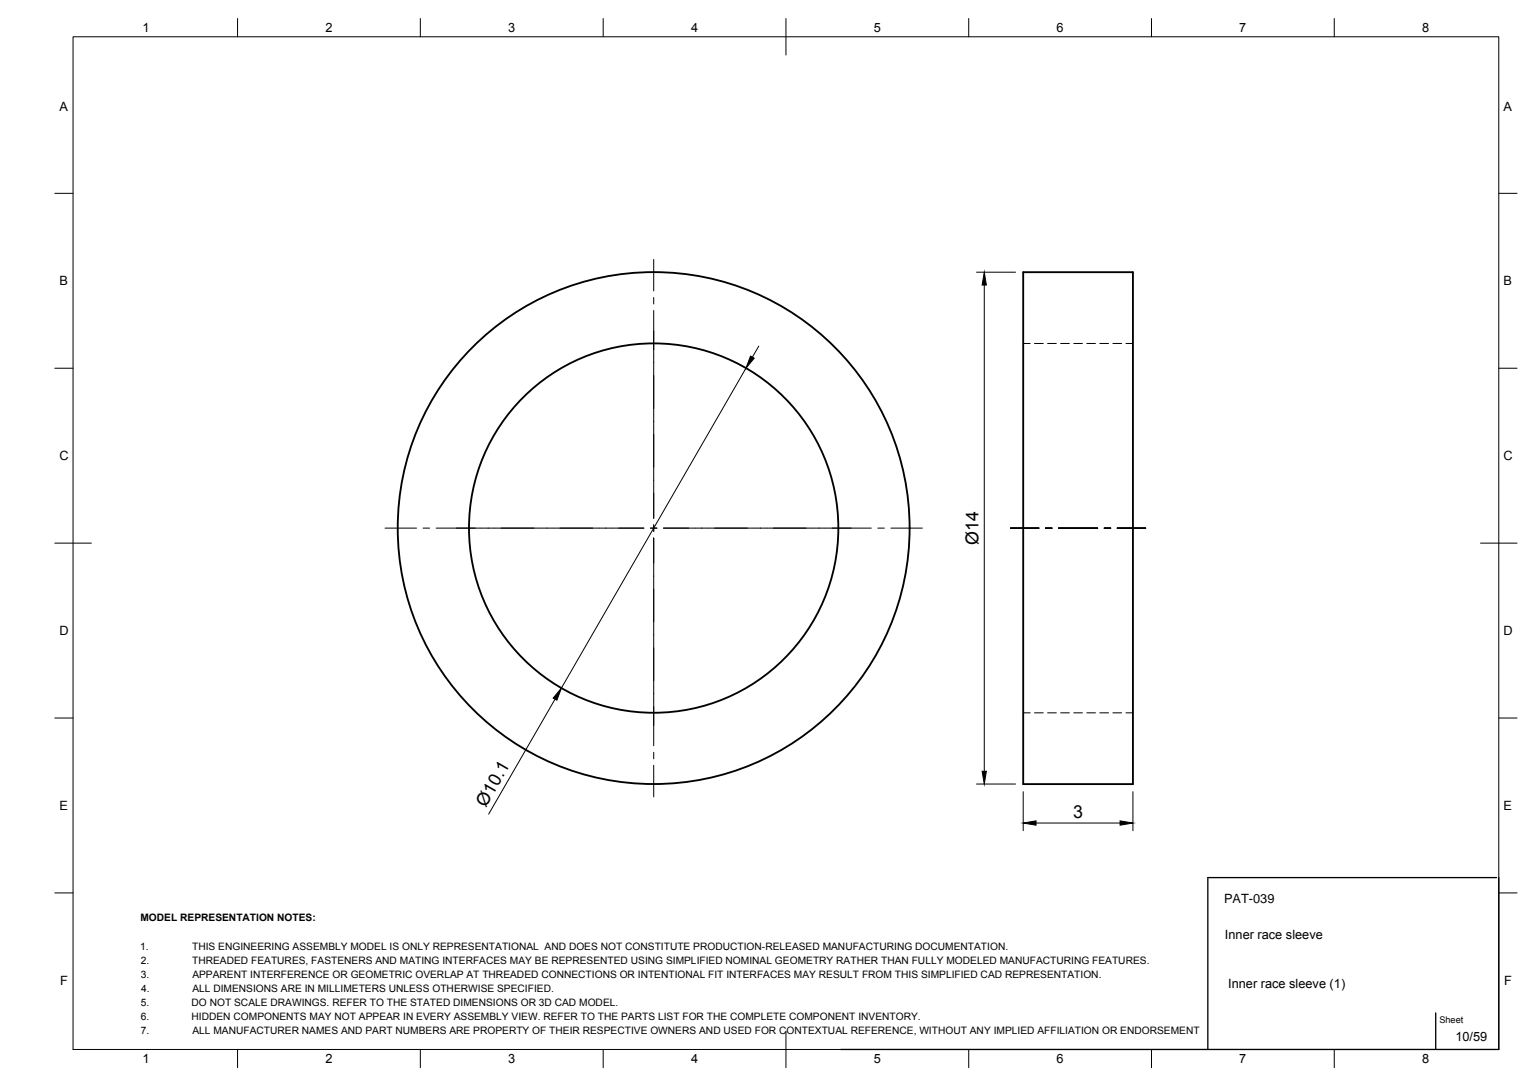
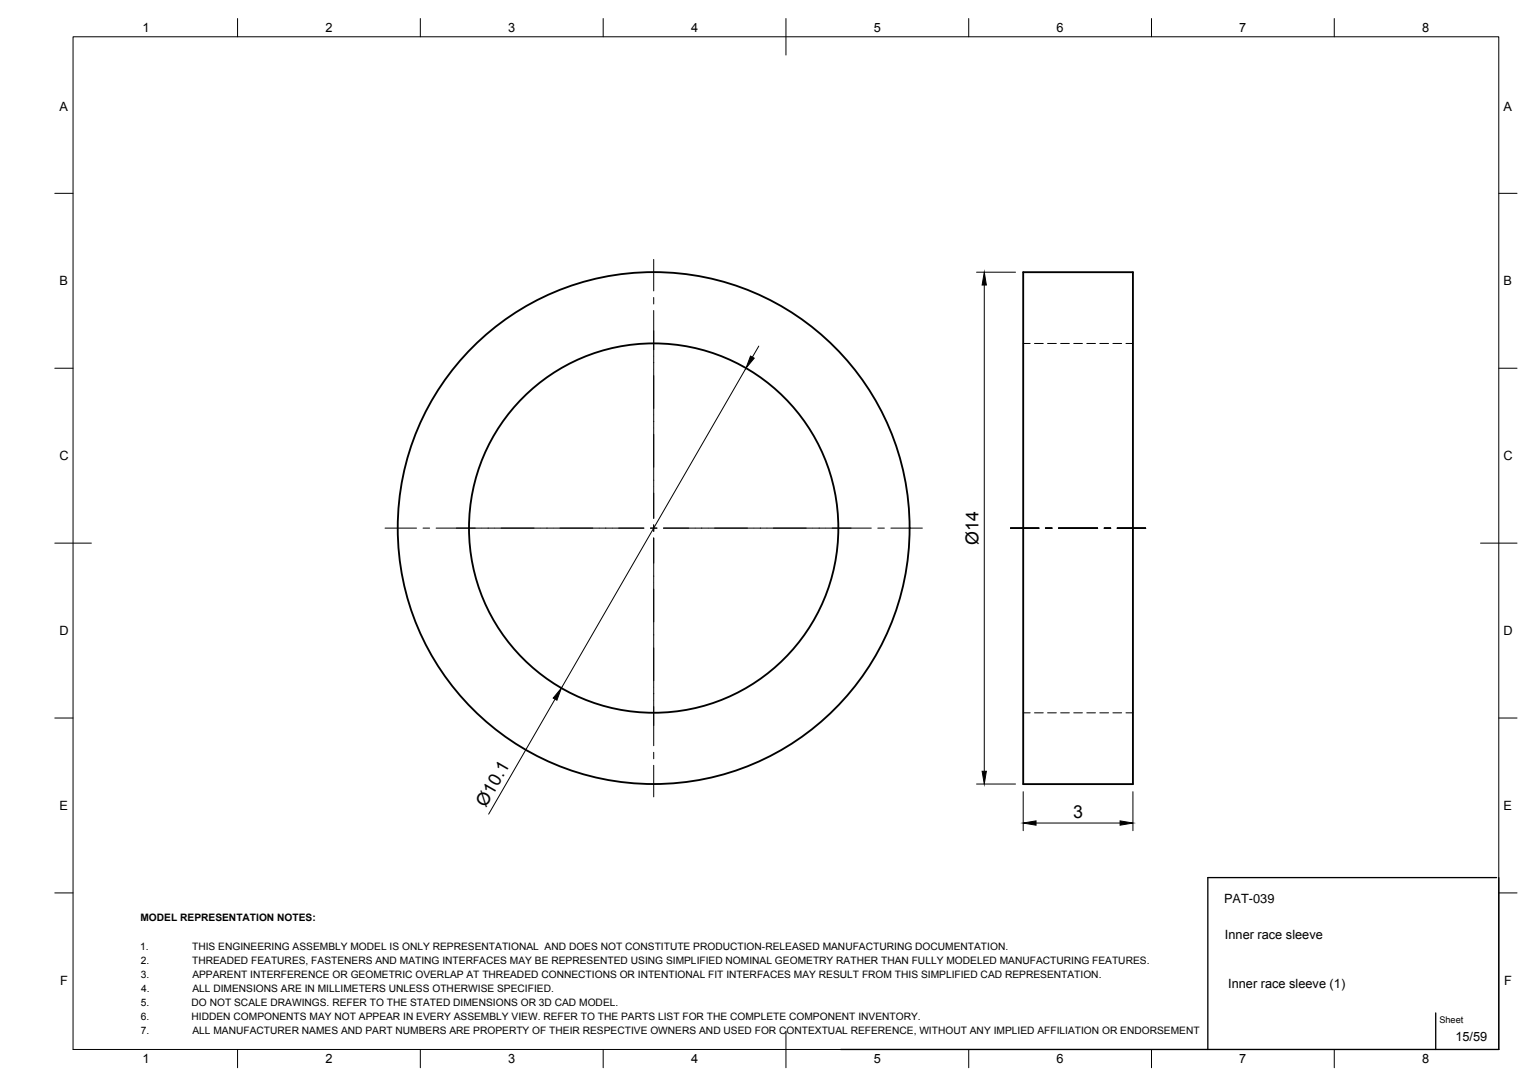
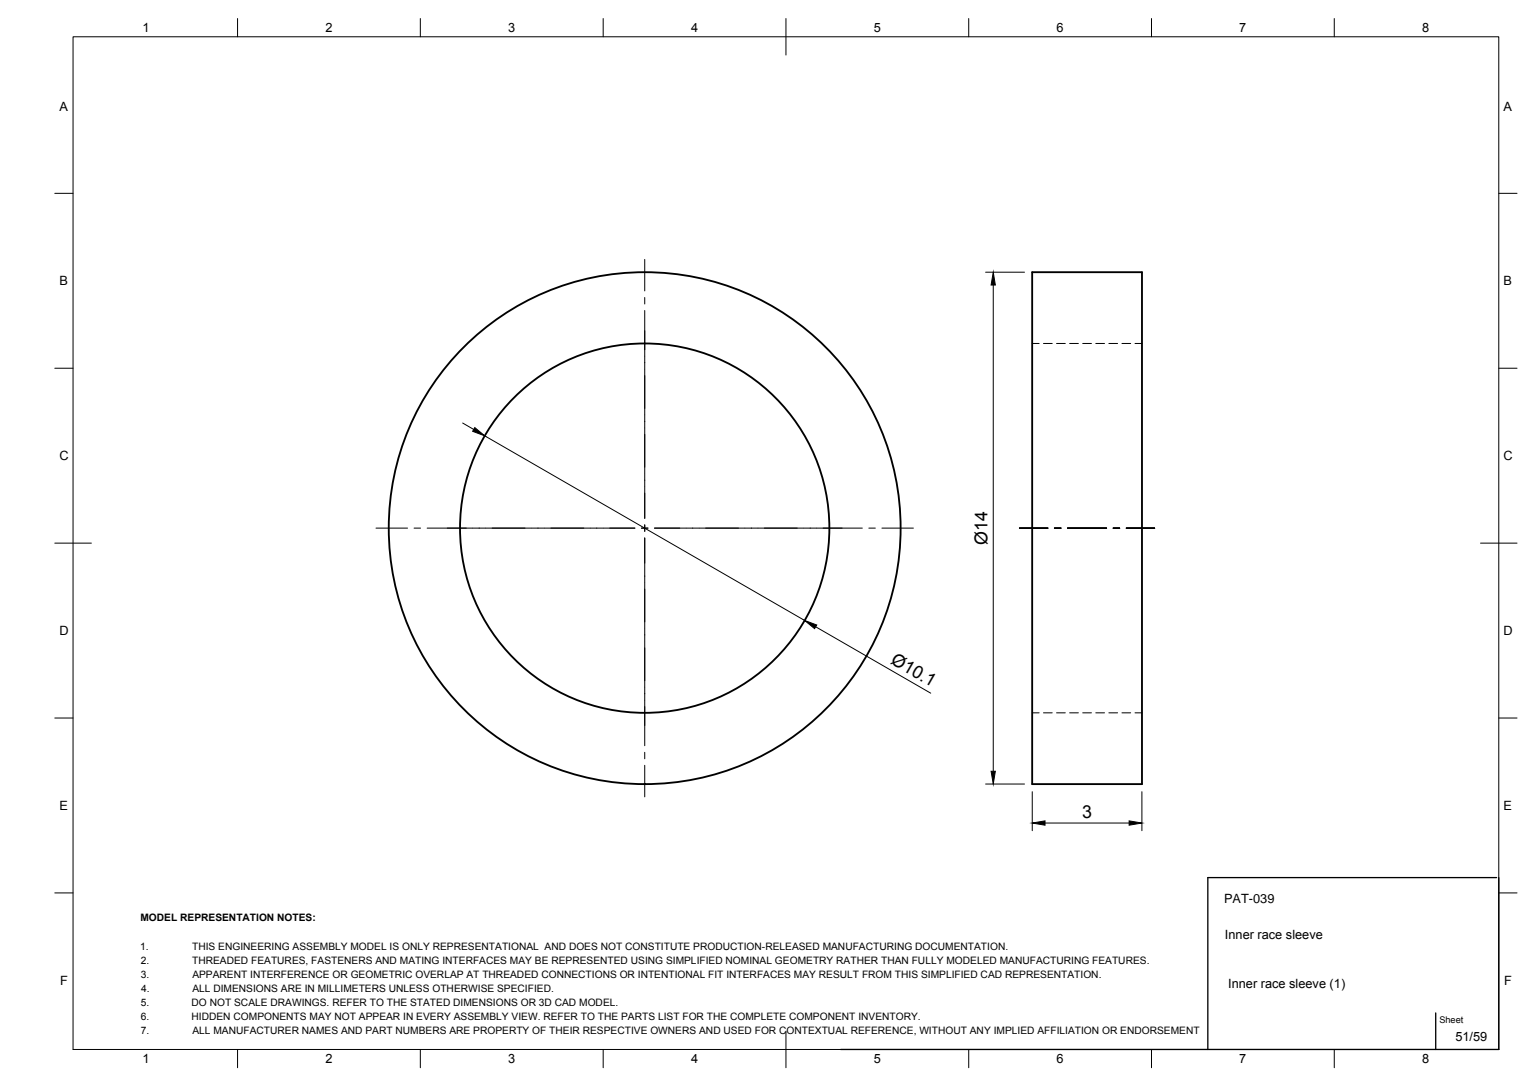
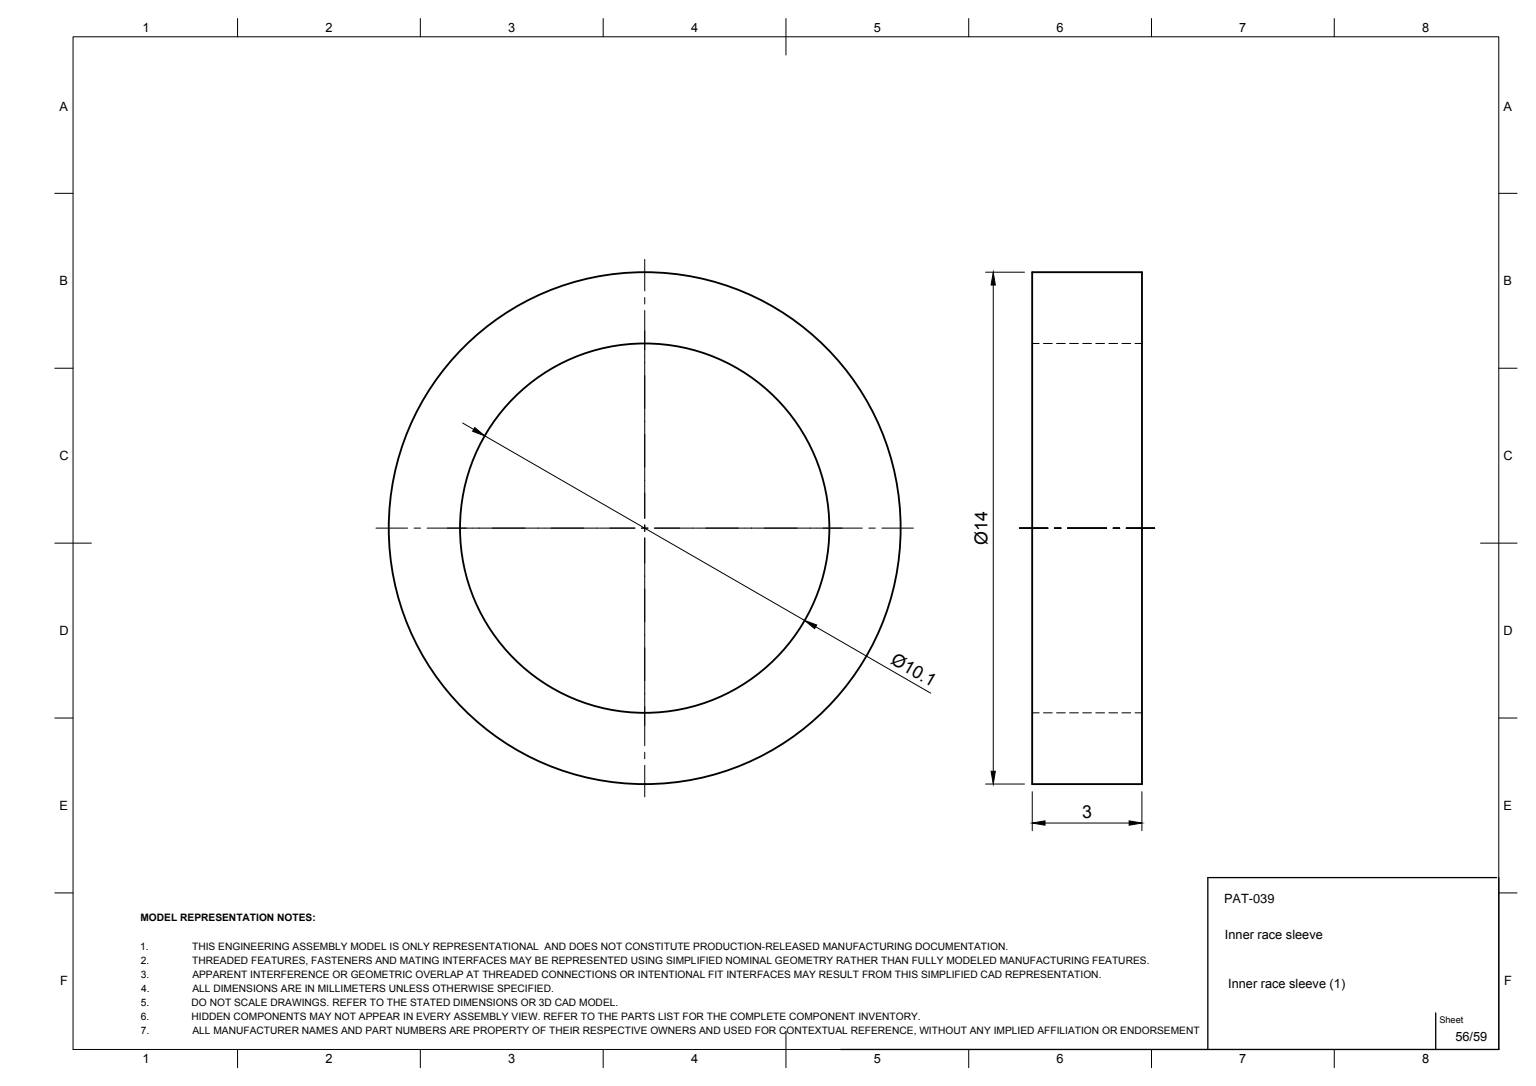
ISO-10303-21;
HEADER;
/* Generated by software containing ST-Developer
 * from STEP Tools, Inc. (www.steptools.com) 
 */

FILE_DESCRIPTION(
/* description */ ('Four-bar parallelogram arm'),
/* implementation_level */ '2;1');

FILE_NAME(
/* name */ 'Inner race sleeve.step',
/* time_stamp */ '2026-10-28T03:24:55-07:00',
/* author */ (''),
/* organization */ (''),
/* preprocessor_version */ 'ST-DEVELOPER v20.2',
/* originating_system */ 'Autodesk Translation Framework v15.17.0.0',
/* authorisation */ '');

FILE_SCHEMA (('AUTOMOTIVE_DESIGN { 1 0 10303 214 3 1 1 }'));
ENDSEC;

DATA;
#10=MECHANICAL_DESIGN_GEOMETRIC_PRESENTATION_REPRESENTATION('',(#627),#14512);
#527=SHAPE_REPRESENTATION_RELATIONSHIP('SRR','None',#14748,#577);
#577=ADVANCED_BREP_SHAPE_REPRESENTATION('',(#685),#14463);
#627=STYLED_ITEM('',(#15087),#685);
#685=MANIFOLD_SOLID_BREP('Body1',#7331);
#777=FACE_BOUND('',#1724,.T.);
#778=FACE_BOUND('',#1726,.T.);
#1040=PLANE('',#8058);
#1041=PLANE('',#8059);
#1259=FACE_OUTER_BOUND('',#1721,.T.);
#1260=FACE_OUTER_BOUND('',#1722,.T.);
#1261=FACE_OUTER_BOUND('',#1723,.T.);
#1262=FACE_OUTER_BOUND('',#1725,.T.);
#1721=EDGE_LOOP('',(#5252,#5253,#5254,#5255));
#1722=EDGE_LOOP('',(#5256,#5257,#5258,#5259));
#1723=EDGE_LOOP('',(#5260));
#1724=EDGE_LOOP('',(#5261));
#1725=EDGE_LOOP('',(#5262));
#1726=EDGE_LOOP('',(#5263));
#2396=LINE('',#11718,#2790);
#2397=LINE('',#11724,#2791);
#2790=VECTOR('',#9286,0.505);
#2791=VECTOR('',#9293,0.7);
#3148=CIRCLE('',#8053,0.505);
#3149=CIRCLE('',#8054,0.505);
#3150=CIRCLE('',#8056,0.7);
#3151=CIRCLE('',#8057,0.7);
#3633=VERTEX_POINT('',#11715);
#3634=VERTEX_POINT('',#11717);
#3635=VERTEX_POINT('',#11721);
#3636=VERTEX_POINT('',#11723);
#4257=EDGE_CURVE('',#3633,#3633,#3148,.T.);
#4258=EDGE_CURVE('',#3633,#3634,#2396,.T.);
#4259=EDGE_CURVE('',#3634,#3634,#3149,.T.);
#4260=EDGE_CURVE('',#3635,#3635,#3150,.T.);
#4261=EDGE_CURVE('',#3635,#3636,#2397,.T.);
#4262=EDGE_CURVE('',#3636,#3636,#3151,.T.);
#5252=ORIENTED_EDGE('',*,*,#4257,.F.);
#5253=ORIENTED_EDGE('',*,*,#4258,.T.);
#5254=ORIENTED_EDGE('',*,*,#4259,.T.);
#5255=ORIENTED_EDGE('',*,*,#4258,.F.);
#5256=ORIENTED_EDGE('',*,*,#4260,.F.);
#5257=ORIENTED_EDGE('',*,*,#4261,.T.);
#5258=ORIENTED_EDGE('',*,*,#4262,.T.);
#5259=ORIENTED_EDGE('',*,*,#4261,.F.);
#5260=ORIENTED_EDGE('',*,*,#4260,.T.);
#5261=ORIENTED_EDGE('',*,*,#4257,.T.);
#5262=ORIENTED_EDGE('',*,*,#4262,.F.);
#5263=ORIENTED_EDGE('',*,*,#4259,.F.);
#6738=CYLINDRICAL_SURFACE('',#8052,0.505);
#6739=CYLINDRICAL_SURFACE('',#8055,0.7);
#6964=ADVANCED_FACE('',(#1259),#6738,.F.);
#6965=ADVANCED_FACE('',(#1260),#6739,.T.);
#6966=ADVANCED_FACE('',(#1261,#777),#1040,.T.);
#6967=ADVANCED_FACE('',(#1262,#778),#1041,.F.);
#7331=CLOSED_SHELL('',(#6964,#6965,#6966,#6967));
#8051=AXIS2_PLACEMENT_3D('',#11713,#9280,#9281);
#8052=AXIS2_PLACEMENT_3D('',#11714,#9282,#9283);
#8053=AXIS2_PLACEMENT_3D('',#11716,#9284,#9285);
#8054=AXIS2_PLACEMENT_3D('',#11719,#9287,#9288);
#8055=AXIS2_PLACEMENT_3D('',#11720,#9289,#9290);
#8056=AXIS2_PLACEMENT_3D('',#11722,#9291,#9292);
#8057=AXIS2_PLACEMENT_3D('',#11725,#9294,#9295);
#8058=AXIS2_PLACEMENT_3D('',#11726,#9296,#9297);
#8059=AXIS2_PLACEMENT_3D('',#11727,#9298,#9299);
#9280=DIRECTION('axis',(0.,0.,1.));
#9281=DIRECTION('refdir',(1.,0.,0.));
#9282=DIRECTION('center_axis',(0.,1.,0.));
#9283=DIRECTION('ref_axis',(1.,0.,0.));
#9284=DIRECTION('center_axis',(0.,-1.,0.));
#9285=DIRECTION('ref_axis',(1.,0.,0.));
#9286=DIRECTION('',(0.,-1.,0.));
#9287=DIRECTION('center_axis',(0.,-1.,0.));
#9288=DIRECTION('ref_axis',(1.,0.,0.));
#9289=DIRECTION('center_axis',(0.,1.,0.));
#9290=DIRECTION('ref_axis',(1.,0.,0.));
#9291=DIRECTION('center_axis',(0.,1.,0.));
#9292=DIRECTION('ref_axis',(1.,0.,0.));
#9293=DIRECTION('',(0.,-1.,0.));
#9294=DIRECTION('center_axis',(0.,1.,0.));
#9295=DIRECTION('ref_axis',(1.,0.,0.));
#9296=DIRECTION('center_axis',(0.,1.,0.));
#9297=DIRECTION('ref_axis',(1.,0.,0.));
#9298=DIRECTION('center_axis',(0.,1.,0.));
#9299=DIRECTION('ref_axis',(1.,0.,0.));
#11713=CARTESIAN_POINT('',(0.,0.,0.));
#11714=CARTESIAN_POINT('Origin',(0.,-0.15,8.));
#11715=CARTESIAN_POINT('',(-0.505,0.15,8.));
#11716=CARTESIAN_POINT('Origin',(0.,0.15,8.));
#11717=CARTESIAN_POINT('',(-0.505,-0.15,8.));
#11718=CARTESIAN_POINT('',(-0.505,-0.15,8.));
#11719=CARTESIAN_POINT('Origin',(0.,-0.15,8.));
#11720=CARTESIAN_POINT('Origin',(0.,-0.15,8.));
#11721=CARTESIAN_POINT('',(-0.7,0.15,8.));
#11722=CARTESIAN_POINT('Origin',(0.,0.15,8.));
#11723=CARTESIAN_POINT('',(-0.7,-0.15,8.));
#11724=CARTESIAN_POINT('',(-0.7,-0.15,8.));
#11725=CARTESIAN_POINT('Origin',(0.,-0.15,8.));
#11726=CARTESIAN_POINT('Origin',(0.,0.15,8.));
#11727=CARTESIAN_POINT('Origin',(0.,-0.15,8.));
#14406=UNCERTAINTY_MEASURE_WITH_UNIT(LENGTH_MEASURE(0.001),#14513,
'DISTANCE_ACCURACY_VALUE',
'Maximum model space distance between geometric entities at asserted c
onnectivities');
#14455=UNCERTAINTY_MEASURE_WITH_UNIT(LENGTH_MEASURE(0.001),#14513,
'DISTANCE_ACCURACY_VALUE',
'Maximum model space distance between geometric entities at asserted c
onnectivities');
#14463=(
GEOMETRIC_REPRESENTATION_CONTEXT(3)
GLOBAL_UNCERTAINTY_ASSIGNED_CONTEXT((#14406))
GLOBAL_UNIT_ASSIGNED_CONTEXT((#14513,#14515,#14516))
REPRESENTATION_CONTEXT('','3D')
);
#14512=(
GEOMETRIC_REPRESENTATION_CONTEXT(3)
GLOBAL_UNCERTAINTY_ASSIGNED_CONTEXT((#14455))
GLOBAL_UNIT_ASSIGNED_CONTEXT((#14513,#14515,#14516))
REPRESENTATION_CONTEXT('','3D')
);
#14513=(
LENGTH_UNIT()
NAMED_UNIT(*)
SI_UNIT(.CENTI.,.METRE.)
);
#14515=(
NAMED_UNIT(*)
PLANE_ANGLE_UNIT()
SI_UNIT($,.RADIAN.)
);
#14516=(
NAMED_UNIT(*)
SI_UNIT($,.STERADIAN.)
SOLID_ANGLE_UNIT()
);
#14524=SHAPE_DEFINITION_REPRESENTATION(#14580,#14748);
#14580=PRODUCT_DEFINITION_SHAPE('',$,#14805);
#14748=SHAPE_REPRESENTATION('',(#8051),#14463);
#14797=PRODUCT_DEFINITION_CONTEXT('part definition',#14967,'design');
#14805=PRODUCT_DEFINITION('Inner race sleeve','Inner race sleeve',#14861,
#14797);
#14861=PRODUCT_DEFINITION_FORMATION('',$,#14976);
#14967=APPLICATION_CONTEXT(
'Core Data for Automotive Mechanical Design Process');
#14968=PRODUCT_CONTEXT('part definition',#14967,'mechanical');
#14976=PRODUCT('Inner race sleeve','Inner race sleeve',
'Inner race sleeve',(#14968));
#15081=COLOUR_RGB('Grey',0.48,0.52,0.57);
#15082=FILL_AREA_STYLE_COLOUR('',#15081);
#15083=FILL_AREA_STYLE('',(#15082));
#15084=SURFACE_STYLE_FILL_AREA(#15083);
#15085=SURFACE_SIDE_STYLE('',(#15084));
#15086=SURFACE_STYLE_USAGE(.BOTH.,#15085);
#15087=PRESENTATION_STYLE_ASSIGNMENT((#15086));
ENDSEC;
END-ISO-10303-21;
